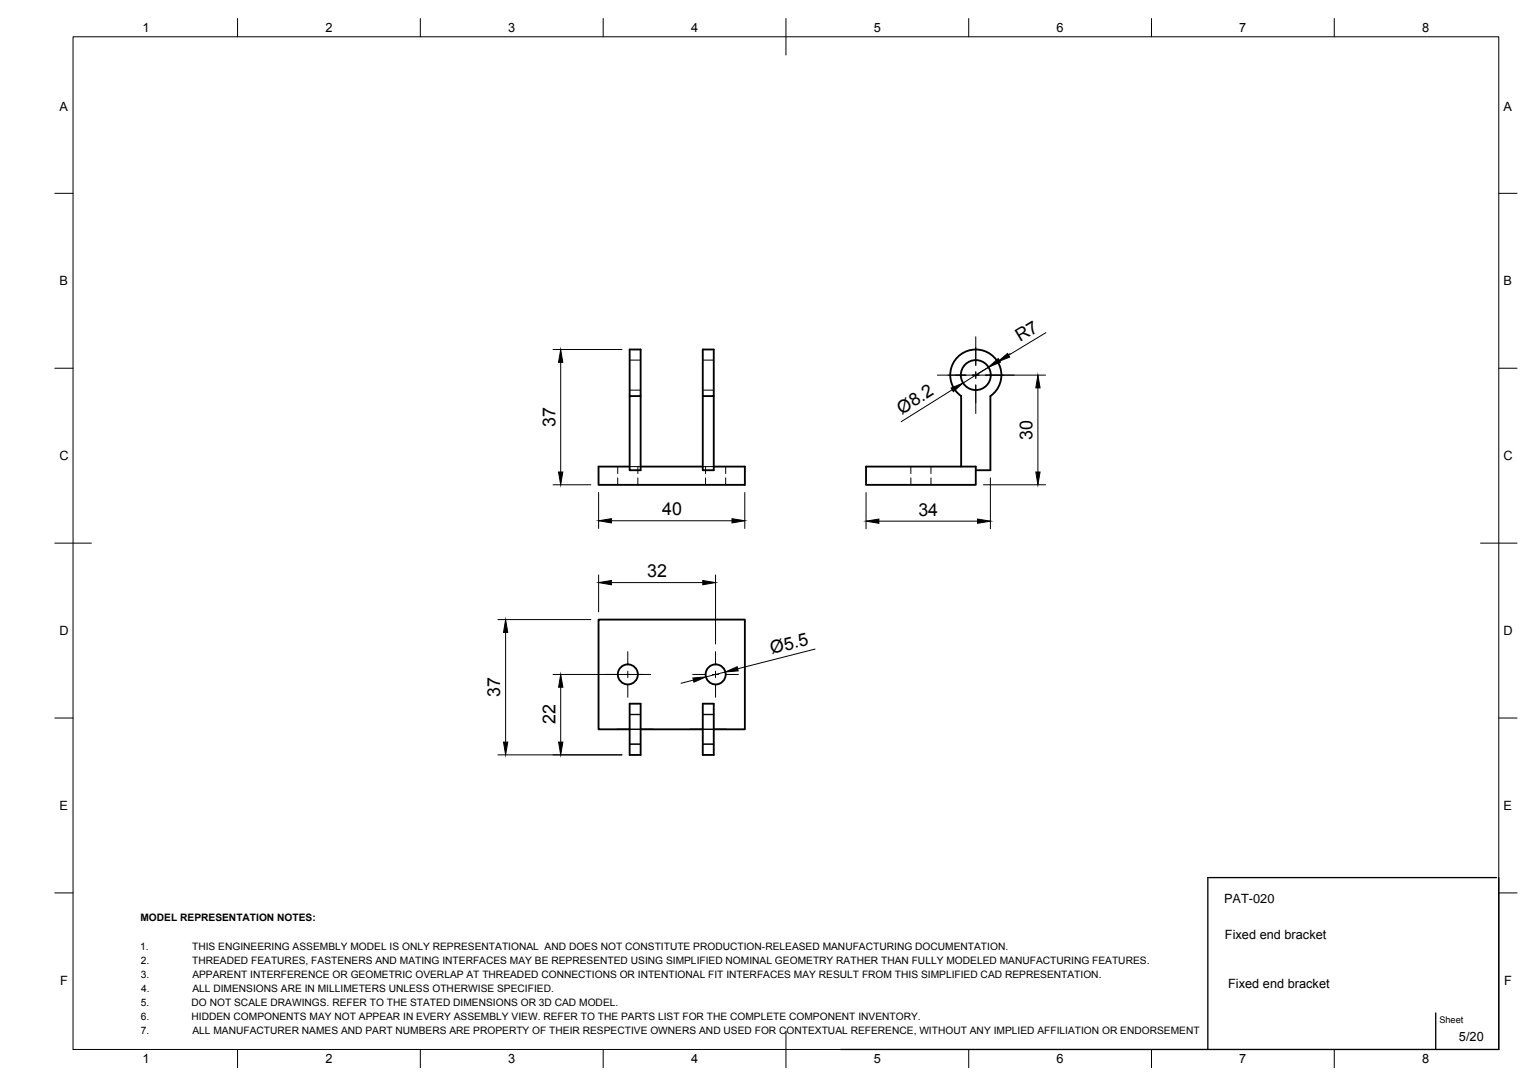
ISO-10303-21;
HEADER;
/* Generated by software containing ST-Developer
 * from STEP Tools, Inc. (www.steptools.com) 
 */

FILE_DESCRIPTION(
/* description */ ('Cable chain and bracket set'),
/* implementation_level */ '2;1');

FILE_NAME(
/* name */ 'Fixed end bracket.step',
/* time_stamp */ '2026-10-29T17:19:47-07:00',
/* author */ (''),
/* organization */ (''),
/* preprocessor_version */ 'ST-DEVELOPER v20.2',
/* originating_system */ 'Autodesk Translation Framework v15.17.0.0',
/* authorisation */ '');

FILE_SCHEMA (('AUTOMOTIVE_DESIGN { 1 0 10303 214 3 1 1 }'));
ENDSEC;

DATA;
#10=MECHANICAL_DESIGN_GEOMETRIC_PRESENTATION_REPRESENTATION('',(#337),#5929);
#311=SHAPE_REPRESENTATION_RELATIONSHIP('SRR','None',#6041,#324);
#324=ADVANCED_BREP_SHAPE_REPRESENTATION('',(#350),#5908);
#337=STYLED_ITEM('',(#6199),#350);
#350=MANIFOLD_SOLID_BREP('Body1',#3331);
#363=FACE_BOUND('',#715,.T.);
#364=FACE_BOUND('',#718,.T.);
#365=FACE_BOUND('',#722,.T.);
#366=FACE_BOUND('',#723,.T.);
#367=FACE_BOUND('',#726,.T.);
#368=FACE_BOUND('',#729,.T.);
#369=FACE_BOUND('',#737,.T.);
#370=FACE_BOUND('',#738,.T.);
#405=PLANE('',#3440);
#406=PLANE('',#3441);
#407=PLANE('',#3442);
#408=PLANE('',#3443);
#409=PLANE('',#3444);
#410=PLANE('',#3445);
#411=PLANE('',#3449);
#412=PLANE('',#3450);
#413=PLANE('',#3451);
#414=PLANE('',#3452);
#415=PLANE('',#3453);
#416=PLANE('',#3454);
#417=PLANE('',#3455);
#418=PLANE('',#3456);
#419=PLANE('',#3457);
#420=PLANE('',#3458);
#527=FACE_OUTER_BOUND('',#709,.T.);
#528=FACE_OUTER_BOUND('',#710,.T.);
#529=FACE_OUTER_BOUND('',#711,.T.);
#530=FACE_OUTER_BOUND('',#712,.T.);
#531=FACE_OUTER_BOUND('',#713,.T.);
#532=FACE_OUTER_BOUND('',#714,.T.);
#533=FACE_OUTER_BOUND('',#716,.T.);
#534=FACE_OUTER_BOUND('',#717,.T.);
#535=FACE_OUTER_BOUND('',#719,.T.);
#536=FACE_OUTER_BOUND('',#720,.T.);
#537=FACE_OUTER_BOUND('',#721,.T.);
#538=FACE_OUTER_BOUND('',#724,.T.);
#539=FACE_OUTER_BOUND('',#725,.T.);
#540=FACE_OUTER_BOUND('',#727,.T.);
#541=FACE_OUTER_BOUND('',#728,.T.);
#542=FACE_OUTER_BOUND('',#730,.T.);
#543=FACE_OUTER_BOUND('',#731,.T.);
#544=FACE_OUTER_BOUND('',#732,.T.);
#545=FACE_OUTER_BOUND('',#733,.T.);
#546=FACE_OUTER_BOUND('',#734,.T.);
#547=FACE_OUTER_BOUND('',#735,.T.);
#548=FACE_OUTER_BOUND('',#736,.T.);
#709=EDGE_LOOP('',(#2249,#2250,#2251,#2252));
#710=EDGE_LOOP('',(#2253,#2254,#2255,#2256));
#711=EDGE_LOOP('',(#2257,#2258,#2259,#2260));
#712=EDGE_LOOP('',(#2261,#2262,#2263,#2264));
#713=EDGE_LOOP('',(#2265,#2266,#2267,#2268));
#714=EDGE_LOOP('',(#2269,#2270,#2271,#2272,#2273,#2274));
#715=EDGE_LOOP('',(#2275));
#716=EDGE_LOOP('',(#2276,#2277,#2278,#2279));
#717=EDGE_LOOP('',(#2280,#2281,#2282,#2283,#2284,#2285));
#718=EDGE_LOOP('',(#2286));
#719=EDGE_LOOP('',(#2287,#2288,#2289,#2290));
#720=EDGE_LOOP('',(#2291,#2292,#2293,#2294));
#721=EDGE_LOOP('',(#2295,#2296,#2297,#2298,#2299,#2300,#2301,#2302,#2303,
#2304,#2305,#2306));
#722=EDGE_LOOP('',(#2307));
#723=EDGE_LOOP('',(#2308));
#724=EDGE_LOOP('',(#2309,#2310,#2311,#2312));
#725=EDGE_LOOP('',(#2313,#2314,#2315,#2316,#2317,#2318));
#726=EDGE_LOOP('',(#2319));
#727=EDGE_LOOP('',(#2320,#2321,#2322,#2323));
#728=EDGE_LOOP('',(#2324,#2325,#2326,#2327,#2328,#2329));
#729=EDGE_LOOP('',(#2330));
#730=EDGE_LOOP('',(#2331,#2332,#2333,#2334));
#731=EDGE_LOOP('',(#2335,#2336,#2337,#2338));
#732=EDGE_LOOP('',(#2339,#2340,#2341,#2342));
#733=EDGE_LOOP('',(#2343,#2344,#2345,#2346,#2347,#2348,#2349,#2350,#2351,
#2352,#2353,#2354));
#734=EDGE_LOOP('',(#2355,#2356,#2357,#2358));
#735=EDGE_LOOP('',(#2359,#2360,#2361,#2362));
#736=EDGE_LOOP('',(#2363,#2364,#2365,#2366));
#737=EDGE_LOOP('',(#2367));
#738=EDGE_LOOP('',(#2368));
#933=LINE('',#4865,#1193);
#934=LINE('',#4871,#1194);
#935=LINE('',#4877,#1195);
#936=LINE('',#4883,#1196);
#937=LINE('',#4888,#1197);
#938=LINE('',#4892,#1198);
#939=LINE('',#4896,#1199);
#940=LINE('',#4898,#1200);
#941=LINE('',#4900,#1201);
#942=LINE('',#4902,#1202);
#943=LINE('',#4903,#1203);
#944=LINE('',#4906,#1204);
#945=LINE('',#4907,#1205);
#946=LINE('',#4910,#1206);
#947=LINE('',#4912,#1207);
#948=LINE('',#4914,#1208);
#949=LINE('',#4915,#1209);
#950=LINE('',#4917,#1210);
#951=LINE('',#4919,#1211);
#952=LINE('',#4922,#1212);
#953=LINE('',#4924,#1213);
#954=LINE('',#4926,#1214);
#955=LINE('',#4928,#1215);
#956=LINE('',#4930,#1216);
#957=LINE('',#4932,#1217);
#958=LINE('',#4934,#1218);
#959=LINE('',#4936,#1219);
#960=LINE('',#4937,#1220);
#961=LINE('',#4941,#1221);
#962=LINE('',#4945,#1222);
#963=LINE('',#4949,#1223);
#964=LINE('',#4951,#1224);
#965=LINE('',#4952,#1225);
#966=LINE('',#4953,#1226);
#967=LINE('',#4956,#1227);
#968=LINE('',#4957,#1228);
#969=LINE('',#4959,#1229);
#970=LINE('',#4961,#1230);
#971=LINE('',#4962,#1231);
#972=LINE('',#4964,#1232);
#973=LINE('',#4969,#1233);
#974=LINE('',#4970,#1234);
#975=LINE('',#4971,#1235);
#976=LINE('',#4974,#1236);
#977=LINE('',#4975,#1237);
#978=LINE('',#4978,#1238);
#979=LINE('',#4979,#1239);
#980=LINE('',#4981,#1240);
#1193=VECTOR('',#3824,0.275);
#1194=VECTOR('',#3831,0.275);
#1195=VECTOR('',#3838,0.41);
#1196=VECTOR('',#3845,0.41);
#1197=VECTOR('',#3850,1.);
#1198=VECTOR('',#3853,1.);
#1199=VECTOR('',#3858,1.);
#1200=VECTOR('',#3859,1.);
#1201=VECTOR('',#3860,1.);
#1202=VECTOR('',#3861,1.);
#1203=VECTOR('',#3862,1.);
#1204=VECTOR('',#3865,1.);
#1205=VECTOR('',#3866,1.);
#1206=VECTOR('',#3869,1.);
#1207=VECTOR('',#3870,1.);
#1208=VECTOR('',#3871,1.);
#1209=VECTOR('',#3872,1.);
#1210=VECTOR('',#3875,1.);
#1211=VECTOR('',#3878,1.);
#1212=VECTOR('',#3881,1.);
#1213=VECTOR('',#3882,1.);
#1214=VECTOR('',#3883,1.);
#1215=VECTOR('',#3884,1.);
#1216=VECTOR('',#3885,1.);
#1217=VECTOR('',#3886,1.);
#1218=VECTOR('',#3887,1.);
#1219=VECTOR('',#3888,1.);
#1220=VECTOR('',#3889,1.);
#1221=VECTOR('',#3892,1.);
#1222=VECTOR('',#3895,1.);
#1223=VECTOR('',#3900,1.);
#1224=VECTOR('',#3901,1.);
#1225=VECTOR('',#3902,1.);
#1226=VECTOR('',#3903,1.);
#1227=VECTOR('',#3906,1.);
#1228=VECTOR('',#3907,1.);
#1229=VECTOR('',#3910,1.);
#1230=VECTOR('',#3911,1.);
#1231=VECTOR('',#3912,1.);
#1232=VECTOR('',#3915,1.);
#1233=VECTOR('',#3920,1.);
#1234=VECTOR('',#3921,1.);
#1235=VECTOR('',#3922,1.);
#1236=VECTOR('',#3925,1.);
#1237=VECTOR('',#3926,1.);
#1238=VECTOR('',#3929,1.);
#1239=VECTOR('',#3930,1.);
#1240=VECTOR('',#3933,1.);
#1453=CIRCLE('',#3426,0.275);
#1454=CIRCLE('',#3427,0.275);
#1455=CIRCLE('',#3429,0.275);
#1456=CIRCLE('',#3430,0.275);
#1457=CIRCLE('',#3432,0.41);
#1458=CIRCLE('',#3433,0.41);
#1459=CIRCLE('',#3435,0.41);
#1460=CIRCLE('',#3436,0.41);
#1461=CIRCLE('',#3438,0.7);
#1462=CIRCLE('',#3439,0.7);
#1463=CIRCLE('',#3447,0.7);
#1464=CIRCLE('',#3448,0.7);
#1561=VERTEX_POINT('',#4862);
#1562=VERTEX_POINT('',#4864);
#1563=VERTEX_POINT('',#4868);
#1564=VERTEX_POINT('',#4870);
#1565=VERTEX_POINT('',#4874);
#1566=VERTEX_POINT('',#4876);
#1567=VERTEX_POINT('',#4880);
#1568=VERTEX_POINT('',#4882);
#1569=VERTEX_POINT('',#4886);
#1570=VERTEX_POINT('',#4887);
#1571=VERTEX_POINT('',#4889);
#1572=VERTEX_POINT('',#4891);
#1573=VERTEX_POINT('',#4895);
#1574=VERTEX_POINT('',#4897);
#1575=VERTEX_POINT('',#4899);
#1576=VERTEX_POINT('',#4901);
#1577=VERTEX_POINT('',#4905);
#1578=VERTEX_POINT('',#4909);
#1579=VERTEX_POINT('',#4911);
#1580=VERTEX_POINT('',#4913);
#1581=VERTEX_POINT('',#4921);
#1582=VERTEX_POINT('',#4923);
#1583=VERTEX_POINT('',#4925);
#1584=VERTEX_POINT('',#4927);
#1585=VERTEX_POINT('',#4929);
#1586=VERTEX_POINT('',#4931);
#1587=VERTEX_POINT('',#4933);
#1588=VERTEX_POINT('',#4935);
#1589=VERTEX_POINT('',#4939);
#1590=VERTEX_POINT('',#4940);
#1591=VERTEX_POINT('',#4942);
#1592=VERTEX_POINT('',#4944);
#1593=VERTEX_POINT('',#4948);
#1594=VERTEX_POINT('',#4950);
#1595=VERTEX_POINT('',#4955);
#1596=VERTEX_POINT('',#4960);
#1597=VERTEX_POINT('',#4967);
#1598=VERTEX_POINT('',#4968);
#1599=VERTEX_POINT('',#4973);
#1600=VERTEX_POINT('',#4977);
#1825=EDGE_CURVE('',#1561,#1561,#1453,.T.);
#1826=EDGE_CURVE('',#1561,#1562,#933,.T.);
#1827=EDGE_CURVE('',#1562,#1562,#1454,.T.);
#1828=EDGE_CURVE('',#1563,#1563,#1455,.T.);
#1829=EDGE_CURVE('',#1563,#1564,#934,.T.);
#1830=EDGE_CURVE('',#1564,#1564,#1456,.T.);
#1831=EDGE_CURVE('',#1565,#1565,#1457,.T.);
#1832=EDGE_CURVE('',#1565,#1566,#935,.T.);
#1833=EDGE_CURVE('',#1566,#1566,#1458,.T.);
#1834=EDGE_CURVE('',#1567,#1567,#1459,.T.);
#1835=EDGE_CURVE('',#1567,#1568,#936,.T.);
#1836=EDGE_CURVE('',#1568,#1568,#1460,.T.);
#1837=EDGE_CURVE('',#1569,#1570,#937,.T.);
#1838=EDGE_CURVE('',#1569,#1571,#1461,.T.);
#1839=EDGE_CURVE('',#1572,#1571,#938,.T.);
#1840=EDGE_CURVE('',#1570,#1572,#1462,.T.);
#1841=EDGE_CURVE('',#1572,#1573,#939,.T.);
#1842=EDGE_CURVE('',#1573,#1574,#940,.T.);
#1843=EDGE_CURVE('',#1575,#1574,#941,.T.);
#1844=EDGE_CURVE('',#1576,#1575,#942,.T.);
#1845=EDGE_CURVE('',#1576,#1570,#943,.T.);
#1846=EDGE_CURVE('',#1577,#1571,#944,.T.);
#1847=EDGE_CURVE('',#1577,#1573,#945,.T.);
#1848=EDGE_CURVE('',#1569,#1578,#946,.T.);
#1849=EDGE_CURVE('',#1579,#1578,#947,.T.);
#1850=EDGE_CURVE('',#1580,#1579,#948,.T.);
#1851=EDGE_CURVE('',#1580,#1577,#949,.T.);
#1852=EDGE_CURVE('',#1574,#1580,#950,.T.);
#1853=EDGE_CURVE('',#1578,#1576,#951,.T.);
#1854=EDGE_CURVE('',#1575,#1581,#952,.T.);
#1855=EDGE_CURVE('',#1581,#1582,#953,.T.);
#1856=EDGE_CURVE('',#1582,#1583,#954,.T.);
#1857=EDGE_CURVE('',#1583,#1584,#955,.T.);
#1858=EDGE_CURVE('',#1584,#1585,#956,.T.);
#1859=EDGE_CURVE('',#1585,#1586,#957,.T.);
#1860=EDGE_CURVE('',#1586,#1587,#958,.T.);
#1861=EDGE_CURVE('',#1587,#1588,#959,.T.);
#1862=EDGE_CURVE('',#1588,#1579,#960,.T.);
#1863=EDGE_CURVE('',#1589,#1590,#961,.T.);
#1864=EDGE_CURVE('',#1589,#1591,#1463,.T.);
#1865=EDGE_CURVE('',#1592,#1591,#962,.T.);
#1866=EDGE_CURVE('',#1590,#1592,#1464,.T.);
#1867=EDGE_CURVE('',#1592,#1593,#963,.T.);
#1868=EDGE_CURVE('',#1593,#1594,#964,.T.);
#1869=EDGE_CURVE('',#1588,#1594,#965,.T.);
#1870=EDGE_CURVE('',#1587,#1590,#966,.T.);
#1871=EDGE_CURVE('',#1595,#1591,#967,.T.);
#1872=EDGE_CURVE('',#1595,#1593,#968,.T.);
#1873=EDGE_CURVE('',#1589,#1586,#969,.T.);
#1874=EDGE_CURVE('',#1596,#1585,#970,.T.);
#1875=EDGE_CURVE('',#1596,#1595,#971,.T.);
#1876=EDGE_CURVE('',#1594,#1596,#972,.T.);
#1877=EDGE_CURVE('',#1597,#1598,#973,.T.);
#1878=EDGE_CURVE('',#1598,#1582,#974,.T.);
#1879=EDGE_CURVE('',#1597,#1581,#975,.T.);
#1880=EDGE_CURVE('',#1599,#1584,#976,.T.);
#1881=EDGE_CURVE('',#1599,#1597,#977,.T.);
#1882=EDGE_CURVE('',#1600,#1599,#978,.T.);
#1883=EDGE_CURVE('',#1600,#1583,#979,.T.);
#1884=EDGE_CURVE('',#1598,#1600,#980,.T.);
#2249=ORIENTED_EDGE('',*,*,#1825,.F.);
#2250=ORIENTED_EDGE('',*,*,#1826,.T.);
#2251=ORIENTED_EDGE('',*,*,#1827,.F.);
#2252=ORIENTED_EDGE('',*,*,#1826,.F.);
#2253=ORIENTED_EDGE('',*,*,#1828,.F.);
#2254=ORIENTED_EDGE('',*,*,#1829,.T.);
#2255=ORIENTED_EDGE('',*,*,#1830,.F.);
#2256=ORIENTED_EDGE('',*,*,#1829,.F.);
#2257=ORIENTED_EDGE('',*,*,#1831,.F.);
#2258=ORIENTED_EDGE('',*,*,#1832,.T.);
#2259=ORIENTED_EDGE('',*,*,#1833,.F.);
#2260=ORIENTED_EDGE('',*,*,#1832,.F.);
#2261=ORIENTED_EDGE('',*,*,#1834,.F.);
#2262=ORIENTED_EDGE('',*,*,#1835,.T.);
#2263=ORIENTED_EDGE('',*,*,#1836,.F.);
#2264=ORIENTED_EDGE('',*,*,#1835,.F.);
#2265=ORIENTED_EDGE('',*,*,#1837,.F.);
#2266=ORIENTED_EDGE('',*,*,#1838,.T.);
#2267=ORIENTED_EDGE('',*,*,#1839,.F.);
#2268=ORIENTED_EDGE('',*,*,#1840,.F.);
#2269=ORIENTED_EDGE('',*,*,#1840,.T.);
#2270=ORIENTED_EDGE('',*,*,#1841,.T.);
#2271=ORIENTED_EDGE('',*,*,#1842,.T.);
#2272=ORIENTED_EDGE('',*,*,#1843,.F.);
#2273=ORIENTED_EDGE('',*,*,#1844,.F.);
#2274=ORIENTED_EDGE('',*,*,#1845,.T.);
#2275=ORIENTED_EDGE('',*,*,#1836,.T.);
#2276=ORIENTED_EDGE('',*,*,#1839,.T.);
#2277=ORIENTED_EDGE('',*,*,#1846,.F.);
#2278=ORIENTED_EDGE('',*,*,#1847,.T.);
#2279=ORIENTED_EDGE('',*,*,#1841,.F.);
#2280=ORIENTED_EDGE('',*,*,#1848,.T.);
#2281=ORIENTED_EDGE('',*,*,#1849,.F.);
#2282=ORIENTED_EDGE('',*,*,#1850,.F.);
#2283=ORIENTED_EDGE('',*,*,#1851,.T.);
#2284=ORIENTED_EDGE('',*,*,#1846,.T.);
#2285=ORIENTED_EDGE('',*,*,#1838,.F.);
#2286=ORIENTED_EDGE('',*,*,#1834,.T.);
#2287=ORIENTED_EDGE('',*,*,#1852,.F.);
#2288=ORIENTED_EDGE('',*,*,#1842,.F.);
#2289=ORIENTED_EDGE('',*,*,#1847,.F.);
#2290=ORIENTED_EDGE('',*,*,#1851,.F.);
#2291=ORIENTED_EDGE('',*,*,#1837,.T.);
#2292=ORIENTED_EDGE('',*,*,#1845,.F.);
#2293=ORIENTED_EDGE('',*,*,#1853,.F.);
#2294=ORIENTED_EDGE('',*,*,#1848,.F.);
#2295=ORIENTED_EDGE('',*,*,#1849,.T.);
#2296=ORIENTED_EDGE('',*,*,#1853,.T.);
#2297=ORIENTED_EDGE('',*,*,#1844,.T.);
#2298=ORIENTED_EDGE('',*,*,#1854,.T.);
#2299=ORIENTED_EDGE('',*,*,#1855,.T.);
#2300=ORIENTED_EDGE('',*,*,#1856,.T.);
#2301=ORIENTED_EDGE('',*,*,#1857,.T.);
#2302=ORIENTED_EDGE('',*,*,#1858,.T.);
#2303=ORIENTED_EDGE('',*,*,#1859,.T.);
#2304=ORIENTED_EDGE('',*,*,#1860,.T.);
#2305=ORIENTED_EDGE('',*,*,#1861,.T.);
#2306=ORIENTED_EDGE('',*,*,#1862,.T.);
#2307=ORIENTED_EDGE('',*,*,#1827,.T.);
#2308=ORIENTED_EDGE('',*,*,#1830,.T.);
#2309=ORIENTED_EDGE('',*,*,#1863,.F.);
#2310=ORIENTED_EDGE('',*,*,#1864,.T.);
#2311=ORIENTED_EDGE('',*,*,#1865,.F.);
#2312=ORIENTED_EDGE('',*,*,#1866,.F.);
#2313=ORIENTED_EDGE('',*,*,#1866,.T.);
#2314=ORIENTED_EDGE('',*,*,#1867,.T.);
#2315=ORIENTED_EDGE('',*,*,#1868,.T.);
#2316=ORIENTED_EDGE('',*,*,#1869,.F.);
#2317=ORIENTED_EDGE('',*,*,#1861,.F.);
#2318=ORIENTED_EDGE('',*,*,#1870,.T.);
#2319=ORIENTED_EDGE('',*,*,#1833,.T.);
#2320=ORIENTED_EDGE('',*,*,#1865,.T.);
#2321=ORIENTED_EDGE('',*,*,#1871,.F.);
#2322=ORIENTED_EDGE('',*,*,#1872,.T.);
#2323=ORIENTED_EDGE('',*,*,#1867,.F.);
#2324=ORIENTED_EDGE('',*,*,#1873,.T.);
#2325=ORIENTED_EDGE('',*,*,#1859,.F.);
#2326=ORIENTED_EDGE('',*,*,#1874,.F.);
#2327=ORIENTED_EDGE('',*,*,#1875,.T.);
#2328=ORIENTED_EDGE('',*,*,#1871,.T.);
#2329=ORIENTED_EDGE('',*,*,#1864,.F.);
#2330=ORIENTED_EDGE('',*,*,#1831,.T.);
#2331=ORIENTED_EDGE('',*,*,#1876,.F.);
#2332=ORIENTED_EDGE('',*,*,#1868,.F.);
#2333=ORIENTED_EDGE('',*,*,#1872,.F.);
#2334=ORIENTED_EDGE('',*,*,#1875,.F.);
#2335=ORIENTED_EDGE('',*,*,#1863,.T.);
#2336=ORIENTED_EDGE('',*,*,#1870,.F.);
#2337=ORIENTED_EDGE('',*,*,#1860,.F.);
#2338=ORIENTED_EDGE('',*,*,#1873,.F.);
#2339=ORIENTED_EDGE('',*,*,#1877,.T.);
#2340=ORIENTED_EDGE('',*,*,#1878,.T.);
#2341=ORIENTED_EDGE('',*,*,#1855,.F.);
#2342=ORIENTED_EDGE('',*,*,#1879,.F.);
#2343=ORIENTED_EDGE('',*,*,#1850,.T.);
#2344=ORIENTED_EDGE('',*,*,#1862,.F.);
#2345=ORIENTED_EDGE('',*,*,#1869,.T.);
#2346=ORIENTED_EDGE('',*,*,#1876,.T.);
#2347=ORIENTED_EDGE('',*,*,#1874,.T.);
#2348=ORIENTED_EDGE('',*,*,#1858,.F.);
#2349=ORIENTED_EDGE('',*,*,#1880,.F.);
#2350=ORIENTED_EDGE('',*,*,#1881,.T.);
#2351=ORIENTED_EDGE('',*,*,#1879,.T.);
#2352=ORIENTED_EDGE('',*,*,#1854,.F.);
#2353=ORIENTED_EDGE('',*,*,#1843,.T.);
#2354=ORIENTED_EDGE('',*,*,#1852,.T.);
#2355=ORIENTED_EDGE('',*,*,#1882,.T.);
#2356=ORIENTED_EDGE('',*,*,#1880,.T.);
#2357=ORIENTED_EDGE('',*,*,#1857,.F.);
#2358=ORIENTED_EDGE('',*,*,#1883,.F.);
#2359=ORIENTED_EDGE('',*,*,#1884,.T.);
#2360=ORIENTED_EDGE('',*,*,#1883,.T.);
#2361=ORIENTED_EDGE('',*,*,#1856,.F.);
#2362=ORIENTED_EDGE('',*,*,#1878,.F.);
#2363=ORIENTED_EDGE('',*,*,#1884,.F.);
#2364=ORIENTED_EDGE('',*,*,#1877,.F.);
#2365=ORIENTED_EDGE('',*,*,#1881,.F.);
#2366=ORIENTED_EDGE('',*,*,#1882,.F.);
#2367=ORIENTED_EDGE('',*,*,#1825,.T.);
#2368=ORIENTED_EDGE('',*,*,#1828,.T.);
#3097=CYLINDRICAL_SURFACE('',#3425,0.275);
#3098=CYLINDRICAL_SURFACE('',#3428,0.275);
#3099=CYLINDRICAL_SURFACE('',#3431,0.41);
#3100=CYLINDRICAL_SURFACE('',#3434,0.41);
#3101=CYLINDRICAL_SURFACE('',#3437,0.7);
#3102=CYLINDRICAL_SURFACE('',#3446,0.7);
#3149=ADVANCED_FACE('',(#527),#3097,.F.);
#3150=ADVANCED_FACE('',(#528),#3098,.F.);
#3151=ADVANCED_FACE('',(#529),#3099,.F.);
#3152=ADVANCED_FACE('',(#530),#3100,.F.);
#3153=ADVANCED_FACE('',(#531),#3101,.T.);
#3154=ADVANCED_FACE('',(#532,#363),#405,.T.);
#3155=ADVANCED_FACE('',(#533),#406,.T.);
#3156=ADVANCED_FACE('',(#534,#364),#407,.F.);
#3157=ADVANCED_FACE('',(#535),#408,.T.);
#3158=ADVANCED_FACE('',(#536),#409,.T.);
#3159=ADVANCED_FACE('',(#537,#365,#366),#410,.T.);
#3160=ADVANCED_FACE('',(#538),#3102,.T.);
#3161=ADVANCED_FACE('',(#539,#367),#411,.T.);
#3162=ADVANCED_FACE('',(#540),#412,.T.);
#3163=ADVANCED_FACE('',(#541,#368),#413,.F.);
#3164=ADVANCED_FACE('',(#542),#414,.T.);
#3165=ADVANCED_FACE('',(#543),#415,.T.);
#3166=ADVANCED_FACE('',(#544),#416,.T.);
#3167=ADVANCED_FACE('',(#545),#417,.T.);
#3168=ADVANCED_FACE('',(#546),#418,.T.);
#3169=ADVANCED_FACE('',(#547),#419,.T.);
#3170=ADVANCED_FACE('',(#548,#369,#370),#420,.F.);
#3331=CLOSED_SHELL('',(#3149,#3150,#3151,#3152,#3153,#3154,#3155,#3156,
#3157,#3158,#3159,#3160,#3161,#3162,#3163,#3164,#3165,#3166,#3167,#3168,
#3169,#3170));
#3424=AXIS2_PLACEMENT_3D('',#4860,#3818,#3819);
#3425=AXIS2_PLACEMENT_3D('',#4861,#3820,#3821);
#3426=AXIS2_PLACEMENT_3D('',#4863,#3822,#3823);
#3427=AXIS2_PLACEMENT_3D('',#4866,#3825,#3826);
#3428=AXIS2_PLACEMENT_3D('',#4867,#3827,#3828);
#3429=AXIS2_PLACEMENT_3D('',#4869,#3829,#3830);
#3430=AXIS2_PLACEMENT_3D('',#4872,#3832,#3833);
#3431=AXIS2_PLACEMENT_3D('',#4873,#3834,#3835);
#3432=AXIS2_PLACEMENT_3D('',#4875,#3836,#3837);
#3433=AXIS2_PLACEMENT_3D('',#4878,#3839,#3840);
#3434=AXIS2_PLACEMENT_3D('',#4879,#3841,#3842);
#3435=AXIS2_PLACEMENT_3D('',#4881,#3843,#3844);
#3436=AXIS2_PLACEMENT_3D('',#4884,#3846,#3847);
#3437=AXIS2_PLACEMENT_3D('',#4885,#3848,#3849);
#3438=AXIS2_PLACEMENT_3D('',#4890,#3851,#3852);
#3439=AXIS2_PLACEMENT_3D('',#4893,#3854,#3855);
#3440=AXIS2_PLACEMENT_3D('',#4894,#3856,#3857);
#3441=AXIS2_PLACEMENT_3D('',#4904,#3863,#3864);
#3442=AXIS2_PLACEMENT_3D('',#4908,#3867,#3868);
#3443=AXIS2_PLACEMENT_3D('',#4916,#3873,#3874);
#3444=AXIS2_PLACEMENT_3D('',#4918,#3876,#3877);
#3445=AXIS2_PLACEMENT_3D('',#4920,#3879,#3880);
#3446=AXIS2_PLACEMENT_3D('',#4938,#3890,#3891);
#3447=AXIS2_PLACEMENT_3D('',#4943,#3893,#3894);
#3448=AXIS2_PLACEMENT_3D('',#4946,#3896,#3897);
#3449=AXIS2_PLACEMENT_3D('',#4947,#3898,#3899);
#3450=AXIS2_PLACEMENT_3D('',#4954,#3904,#3905);
#3451=AXIS2_PLACEMENT_3D('',#4958,#3908,#3909);
#3452=AXIS2_PLACEMENT_3D('',#4963,#3913,#3914);
#3453=AXIS2_PLACEMENT_3D('',#4965,#3916,#3917);
#3454=AXIS2_PLACEMENT_3D('',#4966,#3918,#3919);
#3455=AXIS2_PLACEMENT_3D('',#4972,#3923,#3924);
#3456=AXIS2_PLACEMENT_3D('',#4976,#3927,#3928);
#3457=AXIS2_PLACEMENT_3D('',#4980,#3931,#3932);
#3458=AXIS2_PLACEMENT_3D('',#4982,#3934,#3935);
#3818=DIRECTION('axis',(0.,0.,1.));
#3819=DIRECTION('refdir',(1.,0.,0.));
#3820=DIRECTION('center_axis',(0.,0.,1.));
#3821=DIRECTION('ref_axis',(1.,0.,0.));
#3822=DIRECTION('center_axis',(0.,0.,1.));
#3823=DIRECTION('ref_axis',(1.,0.,0.));
#3824=DIRECTION('',(0.,0.,1.));
#3825=DIRECTION('center_axis',(0.,0.,-1.));
#3826=DIRECTION('ref_axis',(1.,0.,0.));
#3827=DIRECTION('center_axis',(0.,0.,1.));
#3828=DIRECTION('ref_axis',(1.,0.,0.));
#3829=DIRECTION('center_axis',(0.,0.,1.));
#3830=DIRECTION('ref_axis',(1.,0.,0.));
#3831=DIRECTION('',(0.,0.,1.));
#3832=DIRECTION('center_axis',(0.,0.,-1.));
#3833=DIRECTION('ref_axis',(1.,0.,0.));
#3834=DIRECTION('center_axis',(0.,1.,0.));
#3835=DIRECTION('ref_axis',(1.,0.,0.));
#3836=DIRECTION('center_axis',(0.,1.,0.));
#3837=DIRECTION('ref_axis',(1.,0.,0.));
#3838=DIRECTION('',(0.,1.,0.));
#3839=DIRECTION('center_axis',(0.,-1.,0.));
#3840=DIRECTION('ref_axis',(1.,0.,0.));
#3841=DIRECTION('center_axis',(0.,1.,0.));
#3842=DIRECTION('ref_axis',(1.,0.,0.));
#3843=DIRECTION('center_axis',(0.,1.,0.));
#3844=DIRECTION('ref_axis',(1.,0.,0.));
#3845=DIRECTION('',(0.,1.,0.));
#3846=DIRECTION('center_axis',(0.,-1.,0.));
#3847=DIRECTION('ref_axis',(1.,0.,0.));
#3848=DIRECTION('center_axis',(0.,1.,0.));
#3849=DIRECTION('ref_axis',(-1.83697019872103E-16,0.,1.));
#3850=DIRECTION('',(0.,1.,0.));
#3851=DIRECTION('center_axis',(0.,1.,0.));
#3852=DIRECTION('ref_axis',(1.,0.,0.));
#3853=DIRECTION('',(0.,-1.,0.));
#3854=DIRECTION('center_axis',(0.,1.,0.));
#3855=DIRECTION('ref_axis',(1.,0.,0.));
#3856=DIRECTION('center_axis',(0.,1.,0.));
#3857=DIRECTION('ref_axis',(0.,0.,1.));
#3858=DIRECTION('',(0.,0.,-1.));
#3859=DIRECTION('',(-1.,0.,0.));
#3860=DIRECTION('',(0.,0.,-1.));
#3861=DIRECTION('',(1.,0.,0.));
#3862=DIRECTION('',(0.,0.,1.));
#3863=DIRECTION('center_axis',(1.,0.,0.));
#3864=DIRECTION('ref_axis',(0.,0.,-1.));
#3865=DIRECTION('',(0.,0.,1.));
#3866=DIRECTION('',(0.,1.,0.));
#3867=DIRECTION('center_axis',(0.,1.,0.));
#3868=DIRECTION('ref_axis',(1.,0.,0.));
#3869=DIRECTION('',(0.,0.,-1.));
#3870=DIRECTION('',(-1.,0.,0.));
#3871=DIRECTION('',(0.,0.,1.));
#3872=DIRECTION('',(1.,0.,0.));
#3873=DIRECTION('center_axis',(0.,0.,-1.));
#3874=DIRECTION('ref_axis',(-1.,0.,0.));
#3875=DIRECTION('',(0.,-1.,0.));
#3876=DIRECTION('center_axis',(-1.,0.,0.));
#3877=DIRECTION('ref_axis',(0.,0.,1.));
#3878=DIRECTION('',(0.,1.,0.));
#3879=DIRECTION('center_axis',(0.,0.,1.));
#3880=DIRECTION('ref_axis',(1.,0.,0.));
#3881=DIRECTION('',(0.,1.,0.));
#3882=DIRECTION('',(-1.,0.,0.));
#3883=DIRECTION('',(0.,-1.,0.));
#3884=DIRECTION('',(1.,0.,0.));
#3885=DIRECTION('',(0.,1.,0.));
#3886=DIRECTION('',(-1.,0.,0.));
#3887=DIRECTION('',(0.,1.,0.));
#3888=DIRECTION('',(1.,0.,0.));
#3889=DIRECTION('',(0.,1.,0.));
#3890=DIRECTION('center_axis',(0.,1.,0.));
#3891=DIRECTION('ref_axis',(-1.83697019872103E-16,0.,1.));
#3892=DIRECTION('',(0.,1.,0.));
#3893=DIRECTION('center_axis',(0.,1.,0.));
#3894=DIRECTION('ref_axis',(1.,0.,0.));
#3895=DIRECTION('',(0.,-1.,0.));
#3896=DIRECTION('center_axis',(0.,1.,0.));
#3897=DIRECTION('ref_axis',(1.,0.,0.));
#3898=DIRECTION('center_axis',(0.,1.,0.));
#3899=DIRECTION('ref_axis',(0.,0.,1.));
#3900=DIRECTION('',(0.,0.,-1.));
#3901=DIRECTION('',(-1.,0.,0.));
#3902=DIRECTION('',(0.,0.,-1.));
#3903=DIRECTION('',(0.,0.,1.));
#3904=DIRECTION('center_axis',(1.,0.,0.));
#3905=DIRECTION('ref_axis',(0.,0.,-1.));
#3906=DIRECTION('',(0.,0.,1.));
#3907=DIRECTION('',(0.,1.,0.));
#3908=DIRECTION('center_axis',(0.,1.,0.));
#3909=DIRECTION('ref_axis',(1.,0.,0.));
#3910=DIRECTION('',(0.,0.,-1.));
#3911=DIRECTION('',(0.,0.,1.));
#3912=DIRECTION('',(1.,0.,0.));
#3913=DIRECTION('center_axis',(0.,0.,-1.));
#3914=DIRECTION('ref_axis',(-1.,0.,0.));
#3915=DIRECTION('',(0.,-1.,0.));
#3916=DIRECTION('center_axis',(-1.,0.,0.));
#3917=DIRECTION('ref_axis',(0.,0.,1.));
#3918=DIRECTION('center_axis',(0.,1.,0.));
#3919=DIRECTION('ref_axis',(-1.,0.,0.));
#3920=DIRECTION('',(-1.,0.,0.));
#3921=DIRECTION('',(0.,0.,1.));
#3922=DIRECTION('',(0.,0.,1.));
#3923=DIRECTION('center_axis',(1.,0.,0.));
#3924=DIRECTION('ref_axis',(0.,1.,0.));
#3925=DIRECTION('',(0.,0.,1.));
#3926=DIRECTION('',(0.,1.,0.));
#3927=DIRECTION('center_axis',(0.,-1.,0.));
#3928=DIRECTION('ref_axis',(1.,0.,0.));
#3929=DIRECTION('',(1.,0.,0.));
#3930=DIRECTION('',(0.,0.,1.));
#3931=DIRECTION('center_axis',(-1.,0.,0.));
#3932=DIRECTION('ref_axis',(0.,-1.,0.));
#3933=DIRECTION('',(0.,-1.,0.));
#3934=DIRECTION('center_axis',(0.,0.,1.));
#3935=DIRECTION('ref_axis',(1.,0.,0.));
#4860=CARTESIAN_POINT('',(0.,0.,0.));
#4861=CARTESIAN_POINT('Origin',(-1.5,-1.2,-0.1));
#4862=CARTESIAN_POINT('',(-1.775,-1.2,0.));
#4863=CARTESIAN_POINT('Origin',(-1.5,-1.2,0.));
#4864=CARTESIAN_POINT('',(-1.775,-1.2,0.5));
#4865=CARTESIAN_POINT('',(-1.775,-1.2,-0.1));
#4866=CARTESIAN_POINT('Origin',(-1.5,-1.2,0.5));
#4867=CARTESIAN_POINT('Origin',(-1.5,1.2,-0.1));
#4868=CARTESIAN_POINT('',(-1.775,1.2,0.));
#4869=CARTESIAN_POINT('Origin',(-1.5,1.2,0.));
#4870=CARTESIAN_POINT('',(-1.775,1.2,0.5));
#4871=CARTESIAN_POINT('',(-1.775,1.2,-0.1));
#4872=CARTESIAN_POINT('Origin',(-1.5,1.2,0.5));
#4873=CARTESIAN_POINT('Origin',(0.,-1.7,3.));
#4874=CARTESIAN_POINT('',(-0.41,-1.15,3.));
#4875=CARTESIAN_POINT('Origin',(0.,-1.15,3.));
#4876=CARTESIAN_POINT('',(-0.41,-0.85,3.));
#4877=CARTESIAN_POINT('',(-0.41,-1.7,3.));
#4878=CARTESIAN_POINT('Origin',(0.,-0.85,3.));
#4879=CARTESIAN_POINT('Origin',(0.,-1.7,3.));
#4880=CARTESIAN_POINT('',(-0.41,0.85,3.));
#4881=CARTESIAN_POINT('Origin',(0.,0.85,3.));
#4882=CARTESIAN_POINT('',(-0.41,1.15,3.));
#4883=CARTESIAN_POINT('',(-0.41,-1.7,3.));
#4884=CARTESIAN_POINT('Origin',(0.,1.15,3.));
#4885=CARTESIAN_POINT('Origin',(0.,0.85,3.));
#4886=CARTESIAN_POINT('',(-0.4,0.85,2.4255437353462));
#4887=CARTESIAN_POINT('',(-0.4,1.15,2.4255437353462));
#4888=CARTESIAN_POINT('',(-0.4,0.85,2.4255437353462));
#4889=CARTESIAN_POINT('',(0.4,0.85,2.4255437353462));
#4890=CARTESIAN_POINT('Origin',(0.,0.85,3.));
#4891=CARTESIAN_POINT('',(0.4,1.15,2.4255437353462));
#4892=CARTESIAN_POINT('',(0.4,0.85,2.4255437353462));
#4893=CARTESIAN_POINT('Origin',(0.,1.15,3.));
#4894=CARTESIAN_POINT('Origin',(0.,1.15,1.7));
#4895=CARTESIAN_POINT('',(0.4,1.15,0.4));
#4896=CARTESIAN_POINT('',(0.4,1.15,0.4));
#4897=CARTESIAN_POINT('',(0.,1.15,0.4));
#4898=CARTESIAN_POINT('',(-0.4,1.15,0.4));
#4899=CARTESIAN_POINT('',(0.,1.15,0.5));
#4900=CARTESIAN_POINT('',(0.,1.15,0.85));
#4901=CARTESIAN_POINT('',(-0.4,1.15,0.5));
#4902=CARTESIAN_POINT('',(-0.75,1.15,0.5));
#4903=CARTESIAN_POINT('',(-0.4,1.15,3.));
#4904=CARTESIAN_POINT('Origin',(0.4,0.85,3.));
#4905=CARTESIAN_POINT('',(0.4,0.85,0.4));
#4906=CARTESIAN_POINT('',(0.4,0.85,0.4));
#4907=CARTESIAN_POINT('',(0.4,0.85,0.4));
#4908=CARTESIAN_POINT('Origin',(0.,0.85,1.7));
#4909=CARTESIAN_POINT('',(-0.4,0.85,0.5));
#4910=CARTESIAN_POINT('',(-0.4,0.85,3.));
#4911=CARTESIAN_POINT('',(0.,0.85,0.5));
#4912=CARTESIAN_POINT('',(-0.75,0.85,0.5));
#4913=CARTESIAN_POINT('',(0.,0.85,0.4));
#4914=CARTESIAN_POINT('',(0.,0.85,0.85));
#4915=CARTESIAN_POINT('',(-0.4,0.85,0.4));
#4916=CARTESIAN_POINT('Origin',(0.4,0.85,0.4));
#4917=CARTESIAN_POINT('',(0.,-0.575,0.4));
#4918=CARTESIAN_POINT('Origin',(-0.4,0.85,0.4));
#4919=CARTESIAN_POINT('',(-0.4,0.425,0.5));
#4920=CARTESIAN_POINT('Origin',(-1.5,0.,0.5));
#4921=CARTESIAN_POINT('',(0.,2.,0.5));
#4922=CARTESIAN_POINT('',(0.,-2.,0.5));
#4923=CARTESIAN_POINT('',(-3.,2.,0.5));
#4924=CARTESIAN_POINT('',(0.,2.,0.5));
#4925=CARTESIAN_POINT('',(-3.,-2.,0.5));
#4926=CARTESIAN_POINT('',(-3.,2.,0.5));
#4927=CARTESIAN_POINT('',(0.,-2.,0.5));
#4928=CARTESIAN_POINT('',(-3.,-2.,0.5));
#4929=CARTESIAN_POINT('',(0.,-1.15,0.5));
#4930=CARTESIAN_POINT('',(0.,-2.,0.5));
#4931=CARTESIAN_POINT('',(-0.4,-1.15,0.5));
#4932=CARTESIAN_POINT('',(-0.75,-1.15,0.5));
#4933=CARTESIAN_POINT('',(-0.4,-0.85,0.5));
#4934=CARTESIAN_POINT('',(-0.4,-0.575,0.5));
#4935=CARTESIAN_POINT('',(0.,-0.85,0.5));
#4936=CARTESIAN_POINT('',(-0.75,-0.85,0.5));
#4937=CARTESIAN_POINT('',(0.,-2.,0.5));
#4938=CARTESIAN_POINT('Origin',(0.,-1.15,3.));
#4939=CARTESIAN_POINT('',(-0.4,-1.15,2.4255437353462));
#4940=CARTESIAN_POINT('',(-0.4,-0.85,2.4255437353462));
#4941=CARTESIAN_POINT('',(-0.4,-1.15,2.4255437353462));
#4942=CARTESIAN_POINT('',(0.4,-1.15,2.4255437353462));
#4943=CARTESIAN_POINT('Origin',(0.,-1.15,3.));
#4944=CARTESIAN_POINT('',(0.4,-0.85,2.4255437353462));
#4945=CARTESIAN_POINT('',(0.4,-1.15,2.4255437353462));
#4946=CARTESIAN_POINT('Origin',(0.,-0.85,3.));
#4947=CARTESIAN_POINT('Origin',(0.,-0.85,1.7));
#4948=CARTESIAN_POINT('',(0.4,-0.85,0.4));
#4949=CARTESIAN_POINT('',(0.4,-0.85,0.4));
#4950=CARTESIAN_POINT('',(0.,-0.85,0.4));
#4951=CARTESIAN_POINT('',(-0.4,-0.85,0.4));
#4952=CARTESIAN_POINT('',(0.,-0.85,0.85));
#4953=CARTESIAN_POINT('',(-0.4,-0.85,3.));
#4954=CARTESIAN_POINT('Origin',(0.4,-1.15,3.));
#4955=CARTESIAN_POINT('',(0.4,-1.15,0.4));
#4956=CARTESIAN_POINT('',(0.4,-1.15,0.4));
#4957=CARTESIAN_POINT('',(0.4,-1.15,0.4));
#4958=CARTESIAN_POINT('Origin',(0.,-1.15,1.7));
#4959=CARTESIAN_POINT('',(-0.4,-1.15,3.));
#4960=CARTESIAN_POINT('',(0.,-1.15,0.4));
#4961=CARTESIAN_POINT('',(0.,-1.15,0.85));
#4962=CARTESIAN_POINT('',(-0.4,-1.15,0.4));
#4963=CARTESIAN_POINT('Origin',(0.4,-1.15,0.4));
#4964=CARTESIAN_POINT('',(0.,-1.575,0.4));
#4965=CARTESIAN_POINT('Origin',(-0.4,-1.15,0.4));
#4966=CARTESIAN_POINT('Origin',(0.,2.,0.));
#4967=CARTESIAN_POINT('',(0.,2.,0.));
#4968=CARTESIAN_POINT('',(-3.,2.,0.));
#4969=CARTESIAN_POINT('',(0.,2.,0.));
#4970=CARTESIAN_POINT('',(-3.,2.,0.));
#4971=CARTESIAN_POINT('',(0.,2.,0.));
#4972=CARTESIAN_POINT('Origin',(0.,-2.,0.));
#4973=CARTESIAN_POINT('',(0.,-2.,0.));
#4974=CARTESIAN_POINT('',(0.,-2.,0.));
#4975=CARTESIAN_POINT('',(0.,-2.,0.));
#4976=CARTESIAN_POINT('Origin',(-3.,-2.,0.));
#4977=CARTESIAN_POINT('',(-3.,-2.,0.));
#4978=CARTESIAN_POINT('',(-3.,-2.,0.));
#4979=CARTESIAN_POINT('',(-3.,-2.,0.));
#4980=CARTESIAN_POINT('Origin',(-3.,2.,0.));
#4981=CARTESIAN_POINT('',(-3.,2.,0.));
#4982=CARTESIAN_POINT('Origin',(-1.5,0.,0.));
#5884=UNCERTAINTY_MEASURE_WITH_UNIT(LENGTH_MEASURE(0.001),#5930,
'DISTANCE_ACCURACY_VALUE',
'Maximum model space distance between geometric entities at asserted c
onnectivities');
#5905=UNCERTAINTY_MEASURE_WITH_UNIT(LENGTH_MEASURE(0.001),#5930,
'DISTANCE_ACCURACY_VALUE',
'Maximum model space distance between geometric entities at asserted c
onnectivities');
#5908=(
GEOMETRIC_REPRESENTATION_CONTEXT(3)
GLOBAL_UNCERTAINTY_ASSIGNED_CONTEXT((#5884))
GLOBAL_UNIT_ASSIGNED_CONTEXT((#5930,#5932,#5933))
REPRESENTATION_CONTEXT('','3D')
);
#5929=(
GEOMETRIC_REPRESENTATION_CONTEXT(3)
GLOBAL_UNCERTAINTY_ASSIGNED_CONTEXT((#5905))
GLOBAL_UNIT_ASSIGNED_CONTEXT((#5930,#5932,#5933))
REPRESENTATION_CONTEXT('','3D')
);
#5930=(
LENGTH_UNIT()
NAMED_UNIT(*)
SI_UNIT(.CENTI.,.METRE.)
);
#5932=(
NAMED_UNIT(*)
PLANE_ANGLE_UNIT()
SI_UNIT($,.RADIAN.)
);
#5933=(
NAMED_UNIT(*)
SI_UNIT($,.STERADIAN.)
SOLID_ANGLE_UNIT()
);
#5936=SHAPE_DEFINITION_REPRESENTATION(#5959,#6041);
#5959=PRODUCT_DEFINITION_SHAPE('',$,#6065);
#6041=SHAPE_REPRESENTATION('',(#3424),#5908);
#6062=PRODUCT_DEFINITION_CONTEXT('part definition',#6133,'design');
#6065=PRODUCT_DEFINITION('Fixed end bracket','Fixed end bracket',#6088,
#6062);
#6088=PRODUCT_DEFINITION_FORMATION('',$,#6137);
#6133=APPLICATION_CONTEXT(
'Core Data for Automotive Mechanical Design Process');
#6134=PRODUCT_CONTEXT('part definition',#6133,'mechanical');
#6137=PRODUCT('Fixed end bracket','Fixed end bracket',
'Fixed end bracket',(#6134));
#6193=COLOUR_RGB('Dark Blue',0.08,0.2,0.34);
#6194=FILL_AREA_STYLE_COLOUR('',#6193);
#6195=FILL_AREA_STYLE('',(#6194));
#6196=SURFACE_STYLE_FILL_AREA(#6195);
#6197=SURFACE_SIDE_STYLE('',(#6196));
#6198=SURFACE_STYLE_USAGE(.BOTH.,#6197);
#6199=PRESENTATION_STYLE_ASSIGNMENT((#6198));
ENDSEC;
END-ISO-10303-21;
